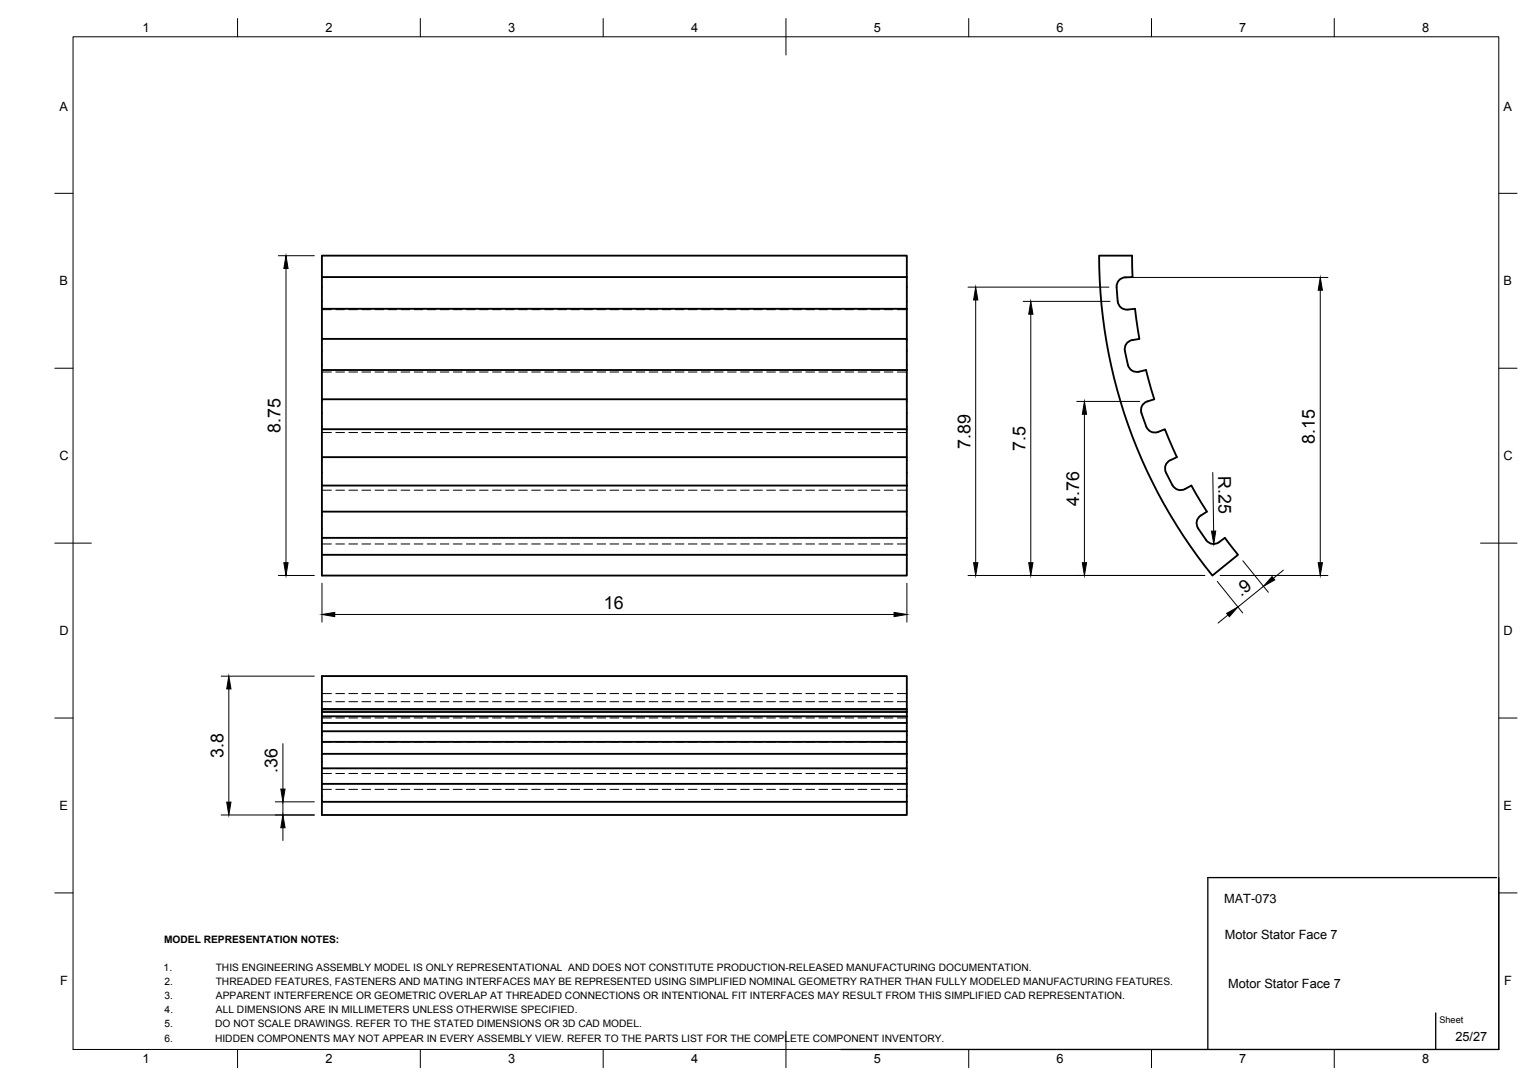
ISO-10303-21;
HEADER;
/* Generated by software containing ST-Developer
 * from STEP Tools, Inc. (www.steptools.com) 
 */

FILE_DESCRIPTION(
/* description */ ('CAx-IF Rec.Pracs.---Representation and Presentation of Product Manufa
cturing Information (PMI)---4.0---2014-10-13'),
/* implementation_level */ '2;1');

FILE_NAME(
/* name */ 'Motor Stator Face 7.step',
/* time_stamp */ '2026-10-24T18:52:33-07:00',
/* author */ (''),
/* organization */ (''),
/* preprocessor_version */ 'ST-DEVELOPER v20.2',
/* originating_system */ 'Autodesk Translation Framework v15.17.0.0',
/* authorisation */ '');

FILE_SCHEMA (('AP242_MANAGED_MODEL_BASED_3D_ENGINEERING_MIM_LF { 1 0 10303 442 2 1 4 }'));
ENDSEC;

DATA;
#10=MECHANICAL_DESIGN_GEOMETRIC_PRESENTATION_REPRESENTATION('',(#442),#34876);
#376=SHAPE_REPRESENTATION_RELATIONSHIP('SRR','None',#35013,#409);
#409=ADVANCED_BREP_SHAPE_REPRESENTATION('',(#475),#34871);
#442=STYLED_ITEM('',(#35162),#475);
#475=MANIFOLD_SOLID_BREP('Motor Stator Face 7',#19582);
#1035=PLANE('',#21978);
#1036=PLANE('',#21988);
#1037=PLANE('',#21998);
#1038=PLANE('',#22008);
#1039=PLANE('',#22018);
#1040=PLANE('',#22019);
#1041=PLANE('',#22020);
#1042=PLANE('',#22021);
#1043=PLANE('',#22022);
#1044=PLANE('',#22029);
#1045=PLANE('',#22039);
#1046=PLANE('',#22042);
#1047=PLANE('',#22045);
#1048=PLANE('',#22048);
#2531=LINE('',#33938,#4130);
#2532=LINE('',#33941,#4131);
#2533=LINE('',#33946,#4132);
#2534=LINE('',#33952,#4133);
#2535=LINE('',#33956,#4134);
#2536=LINE('',#33958,#4135);
#2537=LINE('',#33959,#4136);
#2538=LINE('',#33965,#4137);
#2539=LINE('',#33968,#4138);
#2540=LINE('',#33973,#4139);
#2541=LINE('',#33979,#4140);
#2542=LINE('',#33983,#4141);
#2543=LINE('',#33985,#4142);
#2544=LINE('',#33986,#4143);
#2545=LINE('',#33992,#4144);
#2546=LINE('',#33995,#4145);
#2547=LINE('',#34000,#4146);
#2548=LINE('',#34006,#4147);
#2549=LINE('',#34010,#4148);
#2550=LINE('',#34012,#4149);
#2551=LINE('',#34013,#4150);
#2552=LINE('',#34019,#4151);
#2553=LINE('',#34022,#4152);
#2554=LINE('',#34027,#4153);
#2555=LINE('',#34033,#4154);
#2556=LINE('',#34037,#4155);
#2557=LINE('',#34039,#4156);
#2558=LINE('',#34040,#4157);
#2559=LINE('',#34046,#4158);
#2560=LINE('',#34049,#4159);
#2561=LINE('',#34054,#4160);
#2562=LINE('',#34060,#4161);
#2563=LINE('',#34064,#4162);
#2564=LINE('',#34066,#4163);
#2565=LINE('',#34067,#4164);
#2566=LINE('',#34070,#4165);
#2567=LINE('',#34072,#4166);
#2568=LINE('',#34073,#4167);
#2569=LINE('',#34076,#4168);
#2570=LINE('',#34078,#4169);
#2571=LINE('',#34079,#4170);
#2572=LINE('',#34082,#4171);
#2573=LINE('',#34084,#4172);
#2574=LINE('',#34085,#4173);
#2575=LINE('',#34088,#4174);
#2576=LINE('',#34090,#4175);
#2577=LINE('',#34091,#4176);
#2578=LINE('',#34096,#4177);
#2579=LINE('',#34103,#4178);
#2580=LINE('',#34107,#4179);
#2581=LINE('',#34112,#4180);
#2582=LINE('',#34117,#4181);
#2583=LINE('',#34120,#4182);
#2584=LINE('',#34123,#4183);
#2585=LINE('',#34128,#4184);
#2586=LINE('',#34129,#4185);
#2587=LINE('',#34133,#4186);
#2588=LINE('',#34135,#4187);
#4130=VECTOR('',#27746,1.);
#4131=VECTOR('',#27749,1.);
#4132=VECTOR('',#27754,1.);
#4133=VECTOR('',#27761,1.);
#4134=VECTOR('',#27766,1.);
#4135=VECTOR('',#27767,1.);
#4136=VECTOR('',#27768,1.);
#4137=VECTOR('',#27773,1.);
#4138=VECTOR('',#27776,1.);
#4139=VECTOR('',#27781,1.);
#4140=VECTOR('',#27788,1.);
#4141=VECTOR('',#27793,0.999999999999999);
#4142=VECTOR('',#27794,1.);
#4143=VECTOR('',#27795,0.999999999999999);
#4144=VECTOR('',#27800,1.);
#4145=VECTOR('',#27803,1.);
#4146=VECTOR('',#27808,1.);
#4147=VECTOR('',#27815,1.);
#4148=VECTOR('',#27820,1.);
#4149=VECTOR('',#27821,1.);
#4150=VECTOR('',#27822,1.);
#4151=VECTOR('',#27827,1.);
#4152=VECTOR('',#27830,1.);
#4153=VECTOR('',#27835,1.);
#4154=VECTOR('',#27842,1.);
#4155=VECTOR('',#27847,1.);
#4156=VECTOR('',#27848,1.);
#4157=VECTOR('',#27849,1.);
#4158=VECTOR('',#27854,1.);
#4159=VECTOR('',#27857,1.);
#4160=VECTOR('',#27862,1.);
#4161=VECTOR('',#27869,1.);
#4162=VECTOR('',#27874,1.);
#4163=VECTOR('',#27875,1.);
#4164=VECTOR('',#27876,1.);
#4165=VECTOR('',#27879,1.);
#4166=VECTOR('',#27880,1.);
#4167=VECTOR('',#27881,1.);
#4168=VECTOR('',#27884,0.999999999999999);
#4169=VECTOR('',#27885,1.);
#4170=VECTOR('',#27886,0.999999999999999);
#4171=VECTOR('',#27889,1.);
#4172=VECTOR('',#27890,1.);
#4173=VECTOR('',#27891,1.);
#4174=VECTOR('',#27894,1.);
#4175=VECTOR('',#27895,1.);
#4176=VECTOR('',#27896,1.);
#4177=VECTOR('',#27901,1.);
#4178=VECTOR('',#27912,1.);
#4179=VECTOR('',#27915,1.);
#4180=VECTOR('',#27922,1.);
#4181=VECTOR('',#27929,1.);
#4182=VECTOR('',#27932,1.);
#4183=VECTOR('',#27937,1.);
#4184=VECTOR('',#27944,1.);
#4185=VECTOR('',#27945,1.);
#4186=VECTOR('',#27950,1.);
#4187=VECTOR('',#27953,1.);
#4744=CYLINDRICAL_SURFACE('',#21969,0.00025);
#4745=CYLINDRICAL_SURFACE('',#21972,0.01345);
#4746=CYLINDRICAL_SURFACE('',#21975,0.00025);
#4747=CYLINDRICAL_SURFACE('',#21979,0.00025);
#4748=CYLINDRICAL_SURFACE('',#21982,0.01345);
#4749=CYLINDRICAL_SURFACE('',#21985,0.00025);
#4750=CYLINDRICAL_SURFACE('',#21989,0.00025);
#4751=CYLINDRICAL_SURFACE('',#21992,0.01345);
#4752=CYLINDRICAL_SURFACE('',#21995,0.00025);
#4753=CYLINDRICAL_SURFACE('',#21999,0.00025);
#4754=CYLINDRICAL_SURFACE('',#22002,0.01345);
#4755=CYLINDRICAL_SURFACE('',#22005,0.00025);
#4756=CYLINDRICAL_SURFACE('',#22009,0.00025);
#4757=CYLINDRICAL_SURFACE('',#22012,0.01345);
#4758=CYLINDRICAL_SURFACE('',#22015,0.00025);
#4759=CYLINDRICAL_SURFACE('',#22023,0.013);
#4760=CYLINDRICAL_SURFACE('',#22026,0.013);
#4761=CYLINDRICAL_SURFACE('',#22035,0.013);
#4762=CYLINDRICAL_SURFACE('',#22037,0.013);
#4763=CYLINDRICAL_SURFACE('',#22040,0.013);
#4764=CYLINDRICAL_SURFACE('',#22043,0.0139);
#4765=CYLINDRICAL_SURFACE('',#22046,0.013);
#5721=FACE_OUTER_BOUND('',#6872,.T.);
#5722=FACE_OUTER_BOUND('',#6873,.T.);
#5723=FACE_OUTER_BOUND('',#6874,.T.);
#5724=FACE_OUTER_BOUND('',#6875,.T.);
#5725=FACE_OUTER_BOUND('',#6876,.T.);
#5726=FACE_OUTER_BOUND('',#6877,.T.);
#5727=FACE_OUTER_BOUND('',#6878,.T.);
#5728=FACE_OUTER_BOUND('',#6879,.T.);
#5729=FACE_OUTER_BOUND('',#6880,.T.);
#5730=FACE_OUTER_BOUND('',#6881,.T.);
#5731=FACE_OUTER_BOUND('',#6882,.T.);
#5732=FACE_OUTER_BOUND('',#6883,.T.);
#5733=FACE_OUTER_BOUND('',#6884,.T.);
#5734=FACE_OUTER_BOUND('',#6885,.T.);
#5735=FACE_OUTER_BOUND('',#6886,.T.);
#5736=FACE_OUTER_BOUND('',#6887,.T.);
#5737=FACE_OUTER_BOUND('',#6888,.T.);
#5738=FACE_OUTER_BOUND('',#6889,.T.);
#5739=FACE_OUTER_BOUND('',#6890,.T.);
#5740=FACE_OUTER_BOUND('',#6891,.T.);
#5741=FACE_OUTER_BOUND('',#6892,.T.);
#5742=FACE_OUTER_BOUND('',#6893,.T.);
#5743=FACE_OUTER_BOUND('',#6894,.T.);
#5744=FACE_OUTER_BOUND('',#6895,.T.);
#5745=FACE_OUTER_BOUND('',#6896,.T.);
#5746=FACE_OUTER_BOUND('',#6897,.T.);
#5747=FACE_OUTER_BOUND('',#6898,.T.);
#5748=FACE_OUTER_BOUND('',#6899,.T.);
#5749=FACE_OUTER_BOUND('',#6900,.T.);
#5750=FACE_OUTER_BOUND('',#6901,.T.);
#5751=FACE_OUTER_BOUND('',#6902,.T.);
#5752=FACE_OUTER_BOUND('',#6903,.T.);
#5753=FACE_OUTER_BOUND('',#6904,.T.);
#5754=FACE_OUTER_BOUND('',#6905,.T.);
#5755=FACE_OUTER_BOUND('',#6906,.T.);
#5756=FACE_OUTER_BOUND('',#6907,.T.);
#6872=EDGE_LOOP('',(#17866,#17867,#17868,#17869));
#6873=EDGE_LOOP('',(#17870,#17871,#17872,#17873));
#6874=EDGE_LOOP('',(#17874,#17875,#17876,#17877));
#6875=EDGE_LOOP('',(#17878,#17879,#17880,#17881));
#6876=EDGE_LOOP('',(#17882,#17883,#17884,#17885));
#6877=EDGE_LOOP('',(#17886,#17887,#17888,#17889));
#6878=EDGE_LOOP('',(#17890,#17891,#17892,#17893));
#6879=EDGE_LOOP('',(#17894,#17895,#17896,#17897));
#6880=EDGE_LOOP('',(#17898,#17899,#17900,#17901));
#6881=EDGE_LOOP('',(#17902,#17903,#17904,#17905));
#6882=EDGE_LOOP('',(#17906,#17907,#17908,#17909));
#6883=EDGE_LOOP('',(#17910,#17911,#17912,#17913));
#6884=EDGE_LOOP('',(#17914,#17915,#17916,#17917));
#6885=EDGE_LOOP('',(#17918,#17919,#17920,#17921));
#6886=EDGE_LOOP('',(#17922,#17923,#17924,#17925));
#6887=EDGE_LOOP('',(#17926,#17927,#17928,#17929));
#6888=EDGE_LOOP('',(#17930,#17931,#17932,#17933));
#6889=EDGE_LOOP('',(#17934,#17935,#17936,#17937));
#6890=EDGE_LOOP('',(#17938,#17939,#17940,#17941));
#6891=EDGE_LOOP('',(#17942,#17943,#17944,#17945));
#6892=EDGE_LOOP('',(#17946,#17947,#17948,#17949));
#6893=EDGE_LOOP('',(#17950,#17951,#17952,#17953));
#6894=EDGE_LOOP('',(#17954,#17955,#17956,#17957));
#6895=EDGE_LOOP('',(#17958,#17959,#17960,#17961));
#6896=EDGE_LOOP('',(#17962,#17963,#17964,#17965));
#6897=EDGE_LOOP('',(#17966,#17967,#17968,#17969));
#6898=EDGE_LOOP('',(#17970,#17971,#17972,#17973,#17974,#17975,#17976,#17977,
#17978,#17979,#17980,#17981,#17982,#17983,#17984,#17985,#17986,#17987,#17988,
#17989,#17990,#17991,#17992,#17993,#17994,#17995,#17996,#17997,#17998,#17999,
#18000,#18001,#18002,#18003));
#6899=EDGE_LOOP('',(#18004,#18005,#18006,#18007));
#6900=EDGE_LOOP('',(#18008,#18009,#18010,#18011));
#6901=EDGE_LOOP('',(#18012,#18013,#18014,#18015));
#6902=EDGE_LOOP('',(#18016,#18017,#18018,#18019));
#6903=EDGE_LOOP('',(#18020,#18021,#18022,#18023));
#6904=EDGE_LOOP('',(#18024,#18025,#18026,#18027));
#6905=EDGE_LOOP('',(#18028,#18029,#18030,#18031));
#6906=EDGE_LOOP('',(#18032,#18033,#18034,#18035));
#6907=EDGE_LOOP('',(#18036,#18037,#18038,#18039,#18040,#18041,#18042,#18043,
#18044,#18045,#18046,#18047,#18048,#18049,#18050,#18051,#18052,#18053,#18054,
#18055,#18056,#18057,#18058,#18059,#18060,#18061,#18062,#18063,#18064,#18065,
#18066,#18067,#18068,#18069));
#7941=CIRCLE('',#21970,0.000250000000012414);
#7942=CIRCLE('',#21971,0.000250000000012414);
#7943=CIRCLE('',#21973,0.0134500000000135);
#7944=CIRCLE('',#21974,0.0134500000000135);
#7945=CIRCLE('',#21976,0.000250000000012074);
#7946=CIRCLE('',#21977,0.000250000000012074);
#7947=CIRCLE('',#21980,0.000250000000011423);
#7948=CIRCLE('',#21981,0.000250000000011423);
#7949=CIRCLE('',#21983,0.0134500000000139);
#7950=CIRCLE('',#21984,0.0134500000000139);
#7951=CIRCLE('',#21986,0.00025000000001101);
#7952=CIRCLE('',#21987,0.00025000000001101);
#7953=CIRCLE('',#21990,0.000250000000010237);
#7954=CIRCLE('',#21991,0.000250000000010237);
#7955=CIRCLE('',#21993,0.0134500000000141);
#7956=CIRCLE('',#21994,0.0134500000000141);
#7957=CIRCLE('',#21996,0.000250000000010237);
#7958=CIRCLE('',#21997,0.000250000000010237);
#7959=CIRCLE('',#22000,0.00025000000001101);
#7960=CIRCLE('',#22001,0.00025000000001101);
#7961=CIRCLE('',#22003,0.0134500000000141);
#7962=CIRCLE('',#22004,0.0134500000000141);
#7963=CIRCLE('',#22006,0.000250000000011423);
#7964=CIRCLE('',#22007,0.000250000000011423);
#7965=CIRCLE('',#22010,0.000250000000012074);
#7966=CIRCLE('',#22011,0.000250000000012074);
#7967=CIRCLE('',#22013,0.0134500000000138);
#7968=CIRCLE('',#22014,0.0134500000000138);
#7969=CIRCLE('',#22016,0.000250000000012414);
#7970=CIRCLE('',#22017,0.000250000000012414);
#7971=CIRCLE('',#22024,0.0130000000000133);
#7972=CIRCLE('',#22025,0.0130000000000133);
#7973=CIRCLE('',#22027,0.0130000000000133);
#7974=CIRCLE('',#22028,0.0130000000000133);
#7975=CIRCLE('',#22030,0.0139000000000133);
#7976=CIRCLE('',#22031,0.0130000000000133);
#7977=CIRCLE('',#22032,0.0130000000000133);
#7978=CIRCLE('',#22033,0.0130000000000133);
#7979=CIRCLE('',#22034,0.0130000000000133);
#7980=CIRCLE('',#22036,0.0130000000000133);
#7981=CIRCLE('',#22038,0.0130000000000133);
#7982=CIRCLE('',#22041,0.0130000000000133);
#7983=CIRCLE('',#22044,0.0139000000000133);
#7984=CIRCLE('',#22047,0.0130000000000133);
#9751=VERTEX_POINT('',#33934);
#9752=VERTEX_POINT('',#33935);
#9753=VERTEX_POINT('',#33937);
#9754=VERTEX_POINT('',#33939);
#9755=VERTEX_POINT('',#33943);
#9756=VERTEX_POINT('',#33945);
#9757=VERTEX_POINT('',#33949);
#9758=VERTEX_POINT('',#33951);
#9759=VERTEX_POINT('',#33955);
#9760=VERTEX_POINT('',#33957);
#9761=VERTEX_POINT('',#33961);
#9762=VERTEX_POINT('',#33962);
#9763=VERTEX_POINT('',#33964);
#9764=VERTEX_POINT('',#33966);
#9765=VERTEX_POINT('',#33970);
#9766=VERTEX_POINT('',#33972);
#9767=VERTEX_POINT('',#33976);
#9768=VERTEX_POINT('',#33978);
#9769=VERTEX_POINT('',#33982);
#9770=VERTEX_POINT('',#33984);
#9771=VERTEX_POINT('',#33988);
#9772=VERTEX_POINT('',#33989);
#9773=VERTEX_POINT('',#33991);
#9774=VERTEX_POINT('',#33993);
#9775=VERTEX_POINT('',#33997);
#9776=VERTEX_POINT('',#33999);
#9777=VERTEX_POINT('',#34003);
#9778=VERTEX_POINT('',#34005);
#9779=VERTEX_POINT('',#34009);
#9780=VERTEX_POINT('',#34011);
#9781=VERTEX_POINT('',#34015);
#9782=VERTEX_POINT('',#34016);
#9783=VERTEX_POINT('',#34018);
#9784=VERTEX_POINT('',#34020);
#9785=VERTEX_POINT('',#34024);
#9786=VERTEX_POINT('',#34026);
#9787=VERTEX_POINT('',#34030);
#9788=VERTEX_POINT('',#34032);
#9789=VERTEX_POINT('',#34036);
#9790=VERTEX_POINT('',#34038);
#9791=VERTEX_POINT('',#34042);
#9792=VERTEX_POINT('',#34043);
#9793=VERTEX_POINT('',#34045);
#9794=VERTEX_POINT('',#34047);
#9795=VERTEX_POINT('',#34051);
#9796=VERTEX_POINT('',#34053);
#9797=VERTEX_POINT('',#34057);
#9798=VERTEX_POINT('',#34059);
#9799=VERTEX_POINT('',#34063);
#9800=VERTEX_POINT('',#34065);
#9801=VERTEX_POINT('',#34069);
#9802=VERTEX_POINT('',#34071);
#9803=VERTEX_POINT('',#34075);
#9804=VERTEX_POINT('',#34077);
#9805=VERTEX_POINT('',#34081);
#9806=VERTEX_POINT('',#34083);
#9807=VERTEX_POINT('',#34087);
#9808=VERTEX_POINT('',#34089);
#9809=VERTEX_POINT('',#34093);
#9810=VERTEX_POINT('',#34095);
#9811=VERTEX_POINT('',#34102);
#9812=VERTEX_POINT('',#34104);
#9813=VERTEX_POINT('',#34106);
#9814=VERTEX_POINT('',#34110);
#9815=VERTEX_POINT('',#34115);
#9816=VERTEX_POINT('',#34119);
#9817=VERTEX_POINT('',#34127);
#9818=VERTEX_POINT('',#34131);
#12491=EDGE_CURVE('',#9751,#9752,#7941,.T.);
#12492=EDGE_CURVE('',#9752,#9753,#2531,.T.);
#12493=EDGE_CURVE('',#9753,#9754,#7942,.T.);
#12494=EDGE_CURVE('',#9754,#9751,#2532,.T.);
#12495=EDGE_CURVE('',#9755,#9752,#7943,.T.);
#12496=EDGE_CURVE('',#9756,#9755,#2533,.T.);
#12497=EDGE_CURVE('',#9753,#9756,#7944,.T.);
#12498=EDGE_CURVE('',#9755,#9757,#7945,.T.);
#12499=EDGE_CURVE('',#9757,#9758,#2534,.T.);
#12500=EDGE_CURVE('',#9758,#9756,#7946,.T.);
#12501=EDGE_CURVE('',#9759,#9757,#2535,.T.);
#12502=EDGE_CURVE('',#9760,#9759,#2536,.T.);
#12503=EDGE_CURVE('',#9758,#9760,#2537,.T.);
#12504=EDGE_CURVE('',#9761,#9762,#7947,.T.);
#12505=EDGE_CURVE('',#9762,#9763,#2538,.T.);
#12506=EDGE_CURVE('',#9763,#9764,#7948,.T.);
#12507=EDGE_CURVE('',#9764,#9761,#2539,.T.);
#12508=EDGE_CURVE('',#9765,#9762,#7949,.T.);
#12509=EDGE_CURVE('',#9766,#9765,#2540,.T.);
#12510=EDGE_CURVE('',#9763,#9766,#7950,.T.);
#12511=EDGE_CURVE('',#9765,#9767,#7951,.T.);
#12512=EDGE_CURVE('',#9767,#9768,#2541,.T.);
#12513=EDGE_CURVE('',#9768,#9766,#7952,.T.);
#12514=EDGE_CURVE('',#9769,#9767,#2542,.T.);
#12515=EDGE_CURVE('',#9770,#9769,#2543,.T.);
#12516=EDGE_CURVE('',#9768,#9770,#2544,.T.);
#12517=EDGE_CURVE('',#9771,#9772,#7953,.T.);
#12518=EDGE_CURVE('',#9772,#9773,#2545,.T.);
#12519=EDGE_CURVE('',#9773,#9774,#7954,.T.);
#12520=EDGE_CURVE('',#9774,#9771,#2546,.T.);
#12521=EDGE_CURVE('',#9775,#9772,#7955,.T.);
#12522=EDGE_CURVE('',#9776,#9775,#2547,.T.);
#12523=EDGE_CURVE('',#9773,#9776,#7956,.T.);
#12524=EDGE_CURVE('',#9775,#9777,#7957,.T.);
#12525=EDGE_CURVE('',#9777,#9778,#2548,.T.);
#12526=EDGE_CURVE('',#9778,#9776,#7958,.T.);
#12527=EDGE_CURVE('',#9779,#9777,#2549,.T.);
#12528=EDGE_CURVE('',#9780,#9779,#2550,.T.);
#12529=EDGE_CURVE('',#9778,#9780,#2551,.T.);
#12530=EDGE_CURVE('',#9781,#9782,#7959,.T.);
#12531=EDGE_CURVE('',#9782,#9783,#2552,.T.);
#12532=EDGE_CURVE('',#9783,#9784,#7960,.T.);
#12533=EDGE_CURVE('',#9784,#9781,#2553,.T.);
#12534=EDGE_CURVE('',#9785,#9782,#7961,.T.);
#12535=EDGE_CURVE('',#9786,#9785,#2554,.T.);
#12536=EDGE_CURVE('',#9783,#9786,#7962,.T.);
#12537=EDGE_CURVE('',#9785,#9787,#7963,.T.);
#12538=EDGE_CURVE('',#9787,#9788,#2555,.T.);
#12539=EDGE_CURVE('',#9788,#9786,#7964,.T.);
#12540=EDGE_CURVE('',#9789,#9787,#2556,.T.);
#12541=EDGE_CURVE('',#9790,#9789,#2557,.T.);
#12542=EDGE_CURVE('',#9788,#9790,#2558,.T.);
#12543=EDGE_CURVE('',#9791,#9792,#7965,.T.);
#12544=EDGE_CURVE('',#9792,#9793,#2559,.T.);
#12545=EDGE_CURVE('',#9793,#9794,#7966,.T.);
#12546=EDGE_CURVE('',#9794,#9791,#2560,.T.);
#12547=EDGE_CURVE('',#9795,#9792,#7967,.T.);
#12548=EDGE_CURVE('',#9796,#9795,#2561,.T.);
#12549=EDGE_CURVE('',#9793,#9796,#7968,.T.);
#12550=EDGE_CURVE('',#9795,#9797,#7969,.T.);
#12551=EDGE_CURVE('',#9797,#9798,#2562,.T.);
#12552=EDGE_CURVE('',#9798,#9796,#7970,.T.);
#12553=EDGE_CURVE('',#9799,#9797,#2563,.T.);
#12554=EDGE_CURVE('',#9800,#9799,#2564,.T.);
#12555=EDGE_CURVE('',#9798,#9800,#2565,.T.);
#12556=EDGE_CURVE('',#9801,#9794,#2566,.T.);
#12557=EDGE_CURVE('',#9802,#9801,#2567,.T.);
#12558=EDGE_CURVE('',#9791,#9802,#2568,.T.);
#12559=EDGE_CURVE('',#9803,#9784,#2569,.T.);
#12560=EDGE_CURVE('',#9804,#9803,#2570,.T.);
#12561=EDGE_CURVE('',#9781,#9804,#2571,.T.);
#12562=EDGE_CURVE('',#9805,#9764,#2572,.T.);
#12563=EDGE_CURVE('',#9806,#9805,#2573,.T.);
#12564=EDGE_CURVE('',#9761,#9806,#2574,.T.);
#12565=EDGE_CURVE('',#9807,#9754,#2575,.T.);
#12566=EDGE_CURVE('',#9808,#9807,#2576,.T.);
#12567=EDGE_CURVE('',#9751,#9808,#2577,.T.);
#12568=EDGE_CURVE('',#9809,#9799,#7971,.T.);
#12569=EDGE_CURVE('',#9809,#9810,#2578,.T.);
#12570=EDGE_CURVE('',#9800,#9810,#7972,.T.);
#12571=EDGE_CURVE('',#9780,#9803,#7973,.T.);
#12572=EDGE_CURVE('',#9804,#9779,#7974,.T.);
#12573=EDGE_CURVE('',#9810,#9811,#2579,.T.);
#12574=EDGE_CURVE('',#9811,#9812,#7975,.T.);
#12575=EDGE_CURVE('',#9812,#9813,#2580,.T.);
#12576=EDGE_CURVE('',#9813,#9807,#7976,.T.);
#12577=EDGE_CURVE('',#9760,#9805,#7977,.T.);
#12578=EDGE_CURVE('',#9770,#9814,#7978,.T.);
#12579=EDGE_CURVE('',#9814,#9774,#2581,.T.);
#12580=EDGE_CURVE('',#9790,#9801,#7979,.T.);
#12581=EDGE_CURVE('',#9815,#9769,#7980,.T.);
#12582=EDGE_CURVE('',#9815,#9814,#2582,.T.);
#12583=EDGE_CURVE('',#9813,#9816,#2583,.T.);
#12584=EDGE_CURVE('',#9808,#9816,#7981,.T.);
#12585=EDGE_CURVE('',#9771,#9815,#2584,.T.);
#12586=EDGE_CURVE('',#9802,#9789,#7982,.T.);
#12587=EDGE_CURVE('',#9817,#9809,#2585,.T.);
#12588=EDGE_CURVE('',#9811,#9817,#2586,.T.);
#12589=EDGE_CURVE('',#9818,#9817,#7983,.T.);
#12590=EDGE_CURVE('',#9812,#9818,#2587,.T.);
#12591=EDGE_CURVE('',#9816,#9818,#2588,.T.);
#12592=EDGE_CURVE('',#9806,#9759,#7984,.T.);
#17866=ORIENTED_EDGE('',*,*,#12491,.T.);
#17867=ORIENTED_EDGE('',*,*,#12492,.T.);
#17868=ORIENTED_EDGE('',*,*,#12493,.T.);
#17869=ORIENTED_EDGE('',*,*,#12494,.T.);
#17870=ORIENTED_EDGE('',*,*,#12492,.F.);
#17871=ORIENTED_EDGE('',*,*,#12495,.F.);
#17872=ORIENTED_EDGE('',*,*,#12496,.F.);
#17873=ORIENTED_EDGE('',*,*,#12497,.F.);
#17874=ORIENTED_EDGE('',*,*,#12498,.T.);
#17875=ORIENTED_EDGE('',*,*,#12499,.T.);
#17876=ORIENTED_EDGE('',*,*,#12500,.T.);
#17877=ORIENTED_EDGE('',*,*,#12496,.T.);
#17878=ORIENTED_EDGE('',*,*,#12499,.F.);
#17879=ORIENTED_EDGE('',*,*,#12501,.F.);
#17880=ORIENTED_EDGE('',*,*,#12502,.F.);
#17881=ORIENTED_EDGE('',*,*,#12503,.F.);
#17882=ORIENTED_EDGE('',*,*,#12504,.T.);
#17883=ORIENTED_EDGE('',*,*,#12505,.T.);
#17884=ORIENTED_EDGE('',*,*,#12506,.T.);
#17885=ORIENTED_EDGE('',*,*,#12507,.T.);
#17886=ORIENTED_EDGE('',*,*,#12505,.F.);
#17887=ORIENTED_EDGE('',*,*,#12508,.F.);
#17888=ORIENTED_EDGE('',*,*,#12509,.F.);
#17889=ORIENTED_EDGE('',*,*,#12510,.F.);
#17890=ORIENTED_EDGE('',*,*,#12511,.T.);
#17891=ORIENTED_EDGE('',*,*,#12512,.T.);
#17892=ORIENTED_EDGE('',*,*,#12513,.T.);
#17893=ORIENTED_EDGE('',*,*,#12509,.T.);
#17894=ORIENTED_EDGE('',*,*,#12512,.F.);
#17895=ORIENTED_EDGE('',*,*,#12514,.F.);
#17896=ORIENTED_EDGE('',*,*,#12515,.F.);
#17897=ORIENTED_EDGE('',*,*,#12516,.F.);
#17898=ORIENTED_EDGE('',*,*,#12517,.T.);
#17899=ORIENTED_EDGE('',*,*,#12518,.T.);
#17900=ORIENTED_EDGE('',*,*,#12519,.T.);
#17901=ORIENTED_EDGE('',*,*,#12520,.T.);
#17902=ORIENTED_EDGE('',*,*,#12518,.F.);
#17903=ORIENTED_EDGE('',*,*,#12521,.F.);
#17904=ORIENTED_EDGE('',*,*,#12522,.F.);
#17905=ORIENTED_EDGE('',*,*,#12523,.F.);
#17906=ORIENTED_EDGE('',*,*,#12524,.T.);
#17907=ORIENTED_EDGE('',*,*,#12525,.T.);
#17908=ORIENTED_EDGE('',*,*,#12526,.T.);
#17909=ORIENTED_EDGE('',*,*,#12522,.T.);
#17910=ORIENTED_EDGE('',*,*,#12525,.F.);
#17911=ORIENTED_EDGE('',*,*,#12527,.F.);
#17912=ORIENTED_EDGE('',*,*,#12528,.F.);
#17913=ORIENTED_EDGE('',*,*,#12529,.F.);
#17914=ORIENTED_EDGE('',*,*,#12530,.T.);
#17915=ORIENTED_EDGE('',*,*,#12531,.T.);
#17916=ORIENTED_EDGE('',*,*,#12532,.T.);
#17917=ORIENTED_EDGE('',*,*,#12533,.T.);
#17918=ORIENTED_EDGE('',*,*,#12531,.F.);
#17919=ORIENTED_EDGE('',*,*,#12534,.F.);
#17920=ORIENTED_EDGE('',*,*,#12535,.F.);
#17921=ORIENTED_EDGE('',*,*,#12536,.F.);
#17922=ORIENTED_EDGE('',*,*,#12537,.T.);
#17923=ORIENTED_EDGE('',*,*,#12538,.T.);
#17924=ORIENTED_EDGE('',*,*,#12539,.T.);
#17925=ORIENTED_EDGE('',*,*,#12535,.T.);
#17926=ORIENTED_EDGE('',*,*,#12538,.F.);
#17927=ORIENTED_EDGE('',*,*,#12540,.F.);
#17928=ORIENTED_EDGE('',*,*,#12541,.F.);
#17929=ORIENTED_EDGE('',*,*,#12542,.F.);
#17930=ORIENTED_EDGE('',*,*,#12543,.T.);
#17931=ORIENTED_EDGE('',*,*,#12544,.T.);
#17932=ORIENTED_EDGE('',*,*,#12545,.T.);
#17933=ORIENTED_EDGE('',*,*,#12546,.T.);
#17934=ORIENTED_EDGE('',*,*,#12544,.F.);
#17935=ORIENTED_EDGE('',*,*,#12547,.F.);
#17936=ORIENTED_EDGE('',*,*,#12548,.F.);
#17937=ORIENTED_EDGE('',*,*,#12549,.F.);
#17938=ORIENTED_EDGE('',*,*,#12550,.T.);
#17939=ORIENTED_EDGE('',*,*,#12551,.T.);
#17940=ORIENTED_EDGE('',*,*,#12552,.T.);
#17941=ORIENTED_EDGE('',*,*,#12548,.T.);
#17942=ORIENTED_EDGE('',*,*,#12551,.F.);
#17943=ORIENTED_EDGE('',*,*,#12553,.F.);
#17944=ORIENTED_EDGE('',*,*,#12554,.F.);
#17945=ORIENTED_EDGE('',*,*,#12555,.F.);
#17946=ORIENTED_EDGE('',*,*,#12546,.F.);
#17947=ORIENTED_EDGE('',*,*,#12556,.F.);
#17948=ORIENTED_EDGE('',*,*,#12557,.F.);
#17949=ORIENTED_EDGE('',*,*,#12558,.F.);
#17950=ORIENTED_EDGE('',*,*,#12533,.F.);
#17951=ORIENTED_EDGE('',*,*,#12559,.F.);
#17952=ORIENTED_EDGE('',*,*,#12560,.F.);
#17953=ORIENTED_EDGE('',*,*,#12561,.F.);
#17954=ORIENTED_EDGE('',*,*,#12507,.F.);
#17955=ORIENTED_EDGE('',*,*,#12562,.F.);
#17956=ORIENTED_EDGE('',*,*,#12563,.F.);
#17957=ORIENTED_EDGE('',*,*,#12564,.F.);
#17958=ORIENTED_EDGE('',*,*,#12494,.F.);
#17959=ORIENTED_EDGE('',*,*,#12565,.F.);
#17960=ORIENTED_EDGE('',*,*,#12566,.F.);
#17961=ORIENTED_EDGE('',*,*,#12567,.F.);
#17962=ORIENTED_EDGE('',*,*,#12554,.T.);
#17963=ORIENTED_EDGE('',*,*,#12568,.F.);
#17964=ORIENTED_EDGE('',*,*,#12569,.T.);
#17965=ORIENTED_EDGE('',*,*,#12570,.F.);
#17966=ORIENTED_EDGE('',*,*,#12560,.T.);
#17967=ORIENTED_EDGE('',*,*,#12571,.F.);
#17968=ORIENTED_EDGE('',*,*,#12528,.T.);
#17969=ORIENTED_EDGE('',*,*,#12572,.F.);
#17970=ORIENTED_EDGE('',*,*,#12556,.T.);
#17971=ORIENTED_EDGE('',*,*,#12545,.F.);
#17972=ORIENTED_EDGE('',*,*,#12549,.T.);
#17973=ORIENTED_EDGE('',*,*,#12552,.F.);
#17974=ORIENTED_EDGE('',*,*,#12555,.T.);
#17975=ORIENTED_EDGE('',*,*,#12570,.T.);
#17976=ORIENTED_EDGE('',*,*,#12573,.T.);
#17977=ORIENTED_EDGE('',*,*,#12574,.T.);
#17978=ORIENTED_EDGE('',*,*,#12575,.T.);
#17979=ORIENTED_EDGE('',*,*,#12576,.T.);
#17980=ORIENTED_EDGE('',*,*,#12565,.T.);
#17981=ORIENTED_EDGE('',*,*,#12493,.F.);
#17982=ORIENTED_EDGE('',*,*,#12497,.T.);
#17983=ORIENTED_EDGE('',*,*,#12500,.F.);
#17984=ORIENTED_EDGE('',*,*,#12503,.T.);
#17985=ORIENTED_EDGE('',*,*,#12577,.T.);
#17986=ORIENTED_EDGE('',*,*,#12562,.T.);
#17987=ORIENTED_EDGE('',*,*,#12506,.F.);
#17988=ORIENTED_EDGE('',*,*,#12510,.T.);
#17989=ORIENTED_EDGE('',*,*,#12513,.F.);
#17990=ORIENTED_EDGE('',*,*,#12516,.T.);
#17991=ORIENTED_EDGE('',*,*,#12578,.T.);
#17992=ORIENTED_EDGE('',*,*,#12579,.T.);
#17993=ORIENTED_EDGE('',*,*,#12519,.F.);
#17994=ORIENTED_EDGE('',*,*,#12523,.T.);
#17995=ORIENTED_EDGE('',*,*,#12526,.F.);
#17996=ORIENTED_EDGE('',*,*,#12529,.T.);
#17997=ORIENTED_EDGE('',*,*,#12571,.T.);
#17998=ORIENTED_EDGE('',*,*,#12559,.T.);
#17999=ORIENTED_EDGE('',*,*,#12532,.F.);
#18000=ORIENTED_EDGE('',*,*,#12536,.T.);
#18001=ORIENTED_EDGE('',*,*,#12539,.F.);
#18002=ORIENTED_EDGE('',*,*,#12542,.T.);
#18003=ORIENTED_EDGE('',*,*,#12580,.T.);
#18004=ORIENTED_EDGE('',*,*,#12515,.T.);
#18005=ORIENTED_EDGE('',*,*,#12581,.F.);
#18006=ORIENTED_EDGE('',*,*,#12582,.T.);
#18007=ORIENTED_EDGE('',*,*,#12578,.F.);
#18008=ORIENTED_EDGE('',*,*,#12566,.T.);
#18009=ORIENTED_EDGE('',*,*,#12576,.F.);
#18010=ORIENTED_EDGE('',*,*,#12583,.T.);
#18011=ORIENTED_EDGE('',*,*,#12584,.F.);
#18012=ORIENTED_EDGE('',*,*,#12520,.F.);
#18013=ORIENTED_EDGE('',*,*,#12579,.F.);
#18014=ORIENTED_EDGE('',*,*,#12582,.F.);
#18015=ORIENTED_EDGE('',*,*,#12585,.F.);
#18016=ORIENTED_EDGE('',*,*,#12557,.T.);
#18017=ORIENTED_EDGE('',*,*,#12580,.F.);
#18018=ORIENTED_EDGE('',*,*,#12541,.T.);
#18019=ORIENTED_EDGE('',*,*,#12586,.F.);
#18020=ORIENTED_EDGE('',*,*,#12569,.F.);
#18021=ORIENTED_EDGE('',*,*,#12587,.F.);
#18022=ORIENTED_EDGE('',*,*,#12588,.F.);
#18023=ORIENTED_EDGE('',*,*,#12573,.F.);
#18024=ORIENTED_EDGE('',*,*,#12588,.T.);
#18025=ORIENTED_EDGE('',*,*,#12589,.F.);
#18026=ORIENTED_EDGE('',*,*,#12590,.F.);
#18027=ORIENTED_EDGE('',*,*,#12574,.F.);
#18028=ORIENTED_EDGE('',*,*,#12590,.T.);
#18029=ORIENTED_EDGE('',*,*,#12591,.F.);
#18030=ORIENTED_EDGE('',*,*,#12583,.F.);
#18031=ORIENTED_EDGE('',*,*,#12575,.F.);
#18032=ORIENTED_EDGE('',*,*,#12563,.T.);
#18033=ORIENTED_EDGE('',*,*,#12577,.F.);
#18034=ORIENTED_EDGE('',*,*,#12502,.T.);
#18035=ORIENTED_EDGE('',*,*,#12592,.F.);
#18036=ORIENTED_EDGE('',*,*,#12558,.T.);
#18037=ORIENTED_EDGE('',*,*,#12586,.T.);
#18038=ORIENTED_EDGE('',*,*,#12540,.T.);
#18039=ORIENTED_EDGE('',*,*,#12537,.F.);
#18040=ORIENTED_EDGE('',*,*,#12534,.T.);
#18041=ORIENTED_EDGE('',*,*,#12530,.F.);
#18042=ORIENTED_EDGE('',*,*,#12561,.T.);
#18043=ORIENTED_EDGE('',*,*,#12572,.T.);
#18044=ORIENTED_EDGE('',*,*,#12527,.T.);
#18045=ORIENTED_EDGE('',*,*,#12524,.F.);
#18046=ORIENTED_EDGE('',*,*,#12521,.T.);
#18047=ORIENTED_EDGE('',*,*,#12517,.F.);
#18048=ORIENTED_EDGE('',*,*,#12585,.T.);
#18049=ORIENTED_EDGE('',*,*,#12581,.T.);
#18050=ORIENTED_EDGE('',*,*,#12514,.T.);
#18051=ORIENTED_EDGE('',*,*,#12511,.F.);
#18052=ORIENTED_EDGE('',*,*,#12508,.T.);
#18053=ORIENTED_EDGE('',*,*,#12504,.F.);
#18054=ORIENTED_EDGE('',*,*,#12564,.T.);
#18055=ORIENTED_EDGE('',*,*,#12592,.T.);
#18056=ORIENTED_EDGE('',*,*,#12501,.T.);
#18057=ORIENTED_EDGE('',*,*,#12498,.F.);
#18058=ORIENTED_EDGE('',*,*,#12495,.T.);
#18059=ORIENTED_EDGE('',*,*,#12491,.F.);
#18060=ORIENTED_EDGE('',*,*,#12567,.T.);
#18061=ORIENTED_EDGE('',*,*,#12584,.T.);
#18062=ORIENTED_EDGE('',*,*,#12591,.T.);
#18063=ORIENTED_EDGE('',*,*,#12589,.T.);
#18064=ORIENTED_EDGE('',*,*,#12587,.T.);
#18065=ORIENTED_EDGE('',*,*,#12568,.T.);
#18066=ORIENTED_EDGE('',*,*,#12553,.T.);
#18067=ORIENTED_EDGE('',*,*,#12550,.F.);
#18068=ORIENTED_EDGE('',*,*,#12547,.T.);
#18069=ORIENTED_EDGE('',*,*,#12543,.F.);
#19437=ADVANCED_FACE('',(#5721),#4744,.F.);
#19438=ADVANCED_FACE('',(#5722),#4745,.F.);
#19439=ADVANCED_FACE('',(#5723),#4746,.F.);
#19440=ADVANCED_FACE('',(#5724),#1035,.F.);
#19441=ADVANCED_FACE('',(#5725),#4747,.F.);
#19442=ADVANCED_FACE('',(#5726),#4748,.F.);
#19443=ADVANCED_FACE('',(#5727),#4749,.F.);
#19444=ADVANCED_FACE('',(#5728),#1036,.F.);
#19445=ADVANCED_FACE('',(#5729),#4750,.F.);
#19446=ADVANCED_FACE('',(#5730),#4751,.F.);
#19447=ADVANCED_FACE('',(#5731),#4752,.F.);
#19448=ADVANCED_FACE('',(#5732),#1037,.F.);
#19449=ADVANCED_FACE('',(#5733),#4753,.F.);
#19450=ADVANCED_FACE('',(#5734),#4754,.F.);
#19451=ADVANCED_FACE('',(#5735),#4755,.F.);
#19452=ADVANCED_FACE('',(#5736),#1038,.F.);
#19453=ADVANCED_FACE('',(#5737),#4756,.F.);
#19454=ADVANCED_FACE('',(#5738),#4757,.F.);
#19455=ADVANCED_FACE('',(#5739),#4758,.F.);
#19456=ADVANCED_FACE('',(#5740),#1039,.F.);
#19457=ADVANCED_FACE('',(#5741),#1040,.F.);
#19458=ADVANCED_FACE('',(#5742),#1041,.F.);
#19459=ADVANCED_FACE('',(#5743),#1042,.F.);
#19460=ADVANCED_FACE('',(#5744),#1043,.F.);
#19461=ADVANCED_FACE('',(#5745),#4759,.F.);
#19462=ADVANCED_FACE('',(#5746),#4760,.F.);
#19463=ADVANCED_FACE('',(#5747),#1044,.F.);
#19464=ADVANCED_FACE('',(#5748),#4761,.F.);
#19465=ADVANCED_FACE('',(#5749),#4762,.F.);
#19466=ADVANCED_FACE('',(#5750),#1045,.F.);
#19467=ADVANCED_FACE('',(#5751),#4763,.F.);
#19468=ADVANCED_FACE('',(#5752),#1046,.T.);
#19469=ADVANCED_FACE('',(#5753),#4764,.T.);
#19470=ADVANCED_FACE('',(#5754),#1047,.T.);
#19471=ADVANCED_FACE('',(#5755),#4765,.F.);
#19472=ADVANCED_FACE('',(#5756),#1048,.T.);
#19582=CLOSED_SHELL('',(#19437,#19438,#19439,#19440,#19441,#19442,#19443,
#19444,#19445,#19446,#19447,#19448,#19449,#19450,#19451,#19452,#19453,#19454,
#19455,#19456,#19457,#19458,#19459,#19460,#19461,#19462,#19463,#19464,#19465,
#19466,#19467,#19468,#19469,#19470,#19471,#19472));
#21968=AXIS2_PLACEMENT_3D('',#33932,#27740,#27741);
#21969=AXIS2_PLACEMENT_3D('',#33933,#27742,#27743);
#21970=AXIS2_PLACEMENT_3D('',#33936,#27744,#27745);
#21971=AXIS2_PLACEMENT_3D('',#33940,#27747,#27748);
#21972=AXIS2_PLACEMENT_3D('',#33942,#27750,#27751);
#21973=AXIS2_PLACEMENT_3D('',#33944,#27752,#27753);
#21974=AXIS2_PLACEMENT_3D('',#33947,#27755,#27756);
#21975=AXIS2_PLACEMENT_3D('',#33948,#27757,#27758);
#21976=AXIS2_PLACEMENT_3D('',#33950,#27759,#27760);
#21977=AXIS2_PLACEMENT_3D('',#33953,#27762,#27763);
#21978=AXIS2_PLACEMENT_3D('',#33954,#27764,#27765);
#21979=AXIS2_PLACEMENT_3D('',#33960,#27769,#27770);
#21980=AXIS2_PLACEMENT_3D('',#33963,#27771,#27772);
#21981=AXIS2_PLACEMENT_3D('',#33967,#27774,#27775);
#21982=AXIS2_PLACEMENT_3D('',#33969,#27777,#27778);
#21983=AXIS2_PLACEMENT_3D('',#33971,#27779,#27780);
#21984=AXIS2_PLACEMENT_3D('',#33974,#27782,#27783);
#21985=AXIS2_PLACEMENT_3D('',#33975,#27784,#27785);
#21986=AXIS2_PLACEMENT_3D('',#33977,#27786,#27787);
#21987=AXIS2_PLACEMENT_3D('',#33980,#27789,#27790);
#21988=AXIS2_PLACEMENT_3D('',#33981,#27791,#27792);
#21989=AXIS2_PLACEMENT_3D('',#33987,#27796,#27797);
#21990=AXIS2_PLACEMENT_3D('',#33990,#27798,#27799);
#21991=AXIS2_PLACEMENT_3D('',#33994,#27801,#27802);
#21992=AXIS2_PLACEMENT_3D('',#33996,#27804,#27805);
#21993=AXIS2_PLACEMENT_3D('',#33998,#27806,#27807);
#21994=AXIS2_PLACEMENT_3D('',#34001,#27809,#27810);
#21995=AXIS2_PLACEMENT_3D('',#34002,#27811,#27812);
#21996=AXIS2_PLACEMENT_3D('',#34004,#27813,#27814);
#21997=AXIS2_PLACEMENT_3D('',#34007,#27816,#27817);
#21998=AXIS2_PLACEMENT_3D('',#34008,#27818,#27819);
#21999=AXIS2_PLACEMENT_3D('',#34014,#27823,#27824);
#22000=AXIS2_PLACEMENT_3D('',#34017,#27825,#27826);
#22001=AXIS2_PLACEMENT_3D('',#34021,#27828,#27829);
#22002=AXIS2_PLACEMENT_3D('',#34023,#27831,#27832);
#22003=AXIS2_PLACEMENT_3D('',#34025,#27833,#27834);
#22004=AXIS2_PLACEMENT_3D('',#34028,#27836,#27837);
#22005=AXIS2_PLACEMENT_3D('',#34029,#27838,#27839);
#22006=AXIS2_PLACEMENT_3D('',#34031,#27840,#27841);
#22007=AXIS2_PLACEMENT_3D('',#34034,#27843,#27844);
#22008=AXIS2_PLACEMENT_3D('',#34035,#27845,#27846);
#22009=AXIS2_PLACEMENT_3D('',#34041,#27850,#27851);
#22010=AXIS2_PLACEMENT_3D('',#34044,#27852,#27853);
#22011=AXIS2_PLACEMENT_3D('',#34048,#27855,#27856);
#22012=AXIS2_PLACEMENT_3D('',#34050,#27858,#27859);
#22013=AXIS2_PLACEMENT_3D('',#34052,#27860,#27861);
#22014=AXIS2_PLACEMENT_3D('',#34055,#27863,#27864);
#22015=AXIS2_PLACEMENT_3D('',#34056,#27865,#27866);
#22016=AXIS2_PLACEMENT_3D('',#34058,#27867,#27868);
#22017=AXIS2_PLACEMENT_3D('',#34061,#27870,#27871);
#22018=AXIS2_PLACEMENT_3D('',#34062,#27872,#27873);
#22019=AXIS2_PLACEMENT_3D('',#34068,#27877,#27878);
#22020=AXIS2_PLACEMENT_3D('',#34074,#27882,#27883);
#22021=AXIS2_PLACEMENT_3D('',#34080,#27887,#27888);
#22022=AXIS2_PLACEMENT_3D('',#34086,#27892,#27893);
#22023=AXIS2_PLACEMENT_3D('',#34092,#27897,#27898);
#22024=AXIS2_PLACEMENT_3D('',#34094,#27899,#27900);
#22025=AXIS2_PLACEMENT_3D('',#34097,#27902,#27903);
#22026=AXIS2_PLACEMENT_3D('',#34098,#27904,#27905);
#22027=AXIS2_PLACEMENT_3D('',#34099,#27906,#27907);
#22028=AXIS2_PLACEMENT_3D('',#34100,#27908,#27909);
#22029=AXIS2_PLACEMENT_3D('',#34101,#27910,#27911);
#22030=AXIS2_PLACEMENT_3D('',#34105,#27913,#27914);
#22031=AXIS2_PLACEMENT_3D('',#34108,#27916,#27917);
#22032=AXIS2_PLACEMENT_3D('',#34109,#27918,#27919);
#22033=AXIS2_PLACEMENT_3D('',#34111,#27920,#27921);
#22034=AXIS2_PLACEMENT_3D('',#34113,#27923,#27924);
#22035=AXIS2_PLACEMENT_3D('',#34114,#27925,#27926);
#22036=AXIS2_PLACEMENT_3D('',#34116,#27927,#27928);
#22037=AXIS2_PLACEMENT_3D('',#34118,#27930,#27931);
#22038=AXIS2_PLACEMENT_3D('',#34121,#27933,#27934);
#22039=AXIS2_PLACEMENT_3D('',#34122,#27935,#27936);
#22040=AXIS2_PLACEMENT_3D('',#34124,#27938,#27939);
#22041=AXIS2_PLACEMENT_3D('',#34125,#27940,#27941);
#22042=AXIS2_PLACEMENT_3D('',#34126,#27942,#27943);
#22043=AXIS2_PLACEMENT_3D('',#34130,#27946,#27947);
#22044=AXIS2_PLACEMENT_3D('',#34132,#27948,#27949);
#22045=AXIS2_PLACEMENT_3D('',#34134,#27951,#27952);
#22046=AXIS2_PLACEMENT_3D('',#34136,#27954,#27955);
#22047=AXIS2_PLACEMENT_3D('',#34137,#27956,#27957);
#22048=AXIS2_PLACEMENT_3D('',#34138,#27958,#27959);
#27740=DIRECTION('axis',(0.,0.,1.));
#27741=DIRECTION('refdir',(1.,0.,0.));
#27742=DIRECTION('center_axis',(0.,-1.,0.));
#27743=DIRECTION('ref_axis',(-0.281918008728671,0.,0.95943850055877));
#27744=DIRECTION('center_axis',(0.,1.,0.));
#27745=DIRECTION('ref_axis',(-0.281918008754672,0.,0.95943850055113));
#27746=DIRECTION('',(0.,-1.,0.));
#27747=DIRECTION('center_axis',(0.,-1.,0.));
#27748=DIRECTION('ref_axis',(-0.281918008754672,0.,0.95943850055113));
#27749=DIRECTION('',(0.,1.,0.));
#27750=DIRECTION('center_axis',(0.,-1.,0.));
#27751=DIRECTION('ref_axis',(0.470745247127108,0.,0.882269183586981));
#27752=DIRECTION('center_axis',(0.,-1.,0.));
#27753=DIRECTION('ref_axis',(0.470745247127378,0.,0.882269183586837));
#27754=DIRECTION('',(0.,1.,0.));
#27755=DIRECTION('center_axis',(0.,1.,0.));
#27756=DIRECTION('ref_axis',(0.470745247127378,0.,0.882269183586837));
#27757=DIRECTION('center_axis',(0.,-1.,0.));
#27758=DIRECTION('ref_axis',(0.971857119217081,0.,0.235571092936032));
#27759=DIRECTION('center_axis',(0.,1.,0.));
#27760=DIRECTION('ref_axis',(0.971857119210143,0.,0.235571092964655));
#27761=DIRECTION('',(0.,-1.,0.));
#27762=DIRECTION('center_axis',(0.,-1.,0.));
#27763=DIRECTION('ref_axis',(0.971857119210143,0.,0.235571092964655));
#27764=DIRECTION('center_axis',(0.848811934516349,0.,-0.528694902398929));
#27765=DIRECTION('ref_axis',(0.,-1.,0.));
#27766=DIRECTION('',(0.528694902399201,0.,0.84881193451618));
#27767=DIRECTION('',(0.,1.,0.));
#27768=DIRECTION('',(-0.528694902399201,0.,-0.84881193451618));
#27769=DIRECTION('center_axis',(0.,-1.,0.));
#27770=DIRECTION('ref_axis',(-0.154274306935522,0.,0.9880280553808));
#27771=DIRECTION('center_axis',(0.,1.,0.));
#27772=DIRECTION('ref_axis',(-0.154274306968473,0.,0.988028055375654));
#27773=DIRECTION('',(0.,-1.,0.));
#27774=DIRECTION('center_axis',(0.,-1.,0.));
#27775=DIRECTION('ref_axis',(-0.154274306968473,0.,0.988028055375654));
#27776=DIRECTION('',(0.,1.,0.));
#27777=DIRECTION('center_axis',(0.,-1.,0.));
#27778=DIRECTION('ref_axis',(0.581877193327017,0.,0.813276663802591));
#27779=DIRECTION('center_axis',(0.,-1.,0.));
#27780=DIRECTION('ref_axis',(0.581877193327157,0.,0.813276663802491));
#27781=DIRECTION('',(0.,1.,0.));
#27782=DIRECTION('center_axis',(0.,1.,0.));
#27783=DIRECTION('ref_axis',(0.581877193327157,0.,0.813276663802491));
#27784=DIRECTION('center_axis',(0.,-1.,0.));
#27785=DIRECTION('ref_axis',(0.994290944595386,0.,0.106702940426287));
#27786=DIRECTION('center_axis',(0.,1.,0.));
#27787=DIRECTION('ref_axis',(0.994290944591597,0.,0.106702940461588));
#27788=DIRECTION('',(0.,-1.,0.));
#27789=DIRECTION('center_axis',(0.,-1.,0.));
#27790=DIRECTION('ref_axis',(0.994290944591597,0.,0.106702940461588));
#27791=DIRECTION('center_axis',(0.772541698292714,0.,-0.634964033941301));
#27792=DIRECTION('ref_axis',(0.,-1.,0.));
#27793=DIRECTION('',(0.634964033941407,0.,0.772541698292626));
#27794=DIRECTION('',(0.,1.,0.));
#27795=DIRECTION('',(-0.634964033941407,0.,-0.772541698292626));
#27796=DIRECTION('center_axis',(0.,-1.,0.));
#27797=DIRECTION('ref_axis',(-0.0239909289777986,0.,0.999712176242133));
#27798=DIRECTION('center_axis',(0.,1.,0.));
#27799=DIRECTION('ref_axis',(-0.0239909290168162,0.,0.999712176241197));
#27800=DIRECTION('',(0.,-1.,0.));
#27801=DIRECTION('center_axis',(0.,-1.,0.));
#27802=DIRECTION('ref_axis',(-0.0239909290168162,0.,0.999712176241197));
#27803=DIRECTION('',(0.,1.,0.));
#27804=DIRECTION('center_axis',(0.,-1.,0.));
#27805=DIRECTION('ref_axis',(0.683053059422266,0.,0.730368754817649));
#27806=DIRECTION('center_axis',(0.,-1.,0.));
#27807=DIRECTION('ref_axis',(0.683053059422291,0.,0.730368754817625));
#27808=DIRECTION('',(0.,1.,0.));
#27809=DIRECTION('center_axis',(0.,1.,0.));
#27810=DIRECTION('ref_axis',(0.683053059422291,0.,0.730368754817625));
#27811=DIRECTION('center_axis',(0.,-1.,0.));
#27812=DIRECTION('ref_axis',(0.999712176242133,0.,-0.0239909289777986));
#27813=DIRECTION('center_axis',(0.,1.,0.));
#27814=DIRECTION('ref_axis',(0.999712176241197,0.,-0.0239909290168162));
#27815=DIRECTION('',(0.,-1.,0.));
#27816=DIRECTION('center_axis',(0.,-1.,0.));
#27817=DIRECTION('ref_axis',(0.999712176241197,0.,-0.0239909290168162));
#27818=DIRECTION('center_axis',(0.683053059422266,0.,-0.730368754817649));
#27819=DIRECTION('ref_axis',(0.,-1.,0.));
#27820=DIRECTION('',(0.730368754817616,0.,0.683053059422301));
#27821=DIRECTION('',(0.,1.,0.));
#27822=DIRECTION('',(-0.730368754817616,0.,-0.683053059422301));
#27823=DIRECTION('center_axis',(0.,-1.,0.));
#27824=DIRECTION('ref_axis',(0.106702940426287,0.,0.994290944595386));
#27825=DIRECTION('center_axis',(0.,1.,0.));
#27826=DIRECTION('ref_axis',(0.106702940461588,0.,0.994290944591597));
#27827=DIRECTION('',(0.,-1.,0.));
#27828=DIRECTION('center_axis',(0.,-1.,0.));
#27829=DIRECTION('ref_axis',(0.106702940461588,0.,0.994290944591597));
#27830=DIRECTION('',(0.,1.,0.));
#27831=DIRECTION('center_axis',(0.,-1.,0.));
#27832=DIRECTION('ref_axis',(0.772541698292714,0.,0.634964033941301));
#27833=DIRECTION('center_axis',(0.,-1.,0.));
#27834=DIRECTION('ref_axis',(0.772541698292649,0.,0.63496403394138));
#27835=DIRECTION('',(0.,1.,0.));
#27836=DIRECTION('center_axis',(0.,1.,0.));
#27837=DIRECTION('ref_axis',(0.772541698292649,0.,0.63496403394138));
#27838=DIRECTION('center_axis',(0.,-1.,0.));
#27839=DIRECTION('ref_axis',(0.988028055380798,0.,-0.15427430693553));
#27840=DIRECTION('center_axis',(0.,1.,0.));
#27841=DIRECTION('ref_axis',(0.988028055375653,0.,-0.154274306968481));
#27842=DIRECTION('',(0.,-1.,0.));
#27843=DIRECTION('center_axis',(0.,-1.,0.));
#27844=DIRECTION('ref_axis',(0.988028055375653,0.,-0.154274306968481));
#27845=DIRECTION('center_axis',(0.581877193327018,0.,-0.813276663802591));
#27846=DIRECTION('ref_axis',(0.,-1.,0.));
#27847=DIRECTION('',(0.813276663802457,0.,0.581877193327205));
#27848=DIRECTION('',(0.,1.,0.));
#27849=DIRECTION('',(-0.813276663802457,0.,-0.581877193327205));
#27850=DIRECTION('center_axis',(0.,-1.,0.));
#27851=DIRECTION('ref_axis',(0.235571092936033,0.,0.971857119217081));
#27852=DIRECTION('center_axis',(0.,1.,0.));
#27853=DIRECTION('ref_axis',(0.235571092964656,0.,0.971857119210143));
#27854=DIRECTION('',(0.,-1.,0.));
#27855=DIRECTION('center_axis',(0.,-1.,0.));
#27856=DIRECTION('ref_axis',(0.235571092964656,0.,0.971857119210143));
#27857=DIRECTION('',(0.,1.,0.));
#27858=DIRECTION('center_axis',(0.,-1.,0.));
#27859=DIRECTION('ref_axis',(0.848811934516349,0.,0.528694902398929));
#27860=DIRECTION('center_axis',(0.,-1.,0.));
#27861=DIRECTION('ref_axis',(0.848811934516223,0.,0.528694902399131));
#27862=DIRECTION('',(0.,1.,0.));
#27863=DIRECTION('center_axis',(0.,1.,0.));
#27864=DIRECTION('ref_axis',(0.848811934516223,0.,0.528694902399131));
#27865=DIRECTION('center_axis',(0.,-1.,0.));
#27866=DIRECTION('ref_axis',(0.959438500558773,0.,-0.28191800872866));
#27867=DIRECTION('center_axis',(0.,1.,0.));
#27868=DIRECTION('ref_axis',(0.959438500551133,0.,-0.281918008754661));
#27869=DIRECTION('',(0.,-1.,0.));
#27870=DIRECTION('center_axis',(0.,-1.,0.));
#27871=DIRECTION('ref_axis',(0.959438500551133,0.,-0.281918008754661));
#27872=DIRECTION('center_axis',(0.470745247127108,0.,-0.882269183586981));
#27873=DIRECTION('ref_axis',(0.,-1.,0.));
#27874=DIRECTION('',(0.882269183586787,0.,0.470745247127471));
#27875=DIRECTION('',(0.,1.,0.));
#27876=DIRECTION('',(-0.882269183586787,0.,-0.470745247127471));
#27877=DIRECTION('center_axis',(-0.528694902398929,0.,0.848811934516349));
#27878=DIRECTION('ref_axis',(0.,1.,0.));
#27879=DIRECTION('',(0.84881193451618,0.,0.528694902399201));
#27880=DIRECTION('',(0.,-1.,0.));
#27881=DIRECTION('',(-0.84881193451618,0.,-0.528694902399201));
#27882=DIRECTION('center_axis',(-0.634964033941301,0.,0.772541698292714));
#27883=DIRECTION('ref_axis',(0.,1.,0.));
#27884=DIRECTION('',(0.772541698292626,0.,0.634964033941407));
#27885=DIRECTION('',(0.,-1.,0.));
#27886=DIRECTION('',(-0.772541698292626,0.,-0.634964033941407));
#27887=DIRECTION('center_axis',(-0.813276663802591,0.,0.581877193327018));
#27888=DIRECTION('ref_axis',(0.,1.,0.));
#27889=DIRECTION('',(0.581877193327206,0.,0.813276663802456));
#27890=DIRECTION('',(0.,-1.,0.));
#27891=DIRECTION('',(-0.581877193327206,0.,-0.813276663802456));
#27892=DIRECTION('center_axis',(-0.882269183586981,0.,0.470745247127108));
#27893=DIRECTION('ref_axis',(0.,1.,0.));
#27894=DIRECTION('',(0.470745247127471,0.,0.882269183586787));
#27895=DIRECTION('',(0.,-1.,0.));
#27896=DIRECTION('',(-0.470745247127471,0.,-0.882269183586787));
#27897=DIRECTION('center_axis',(0.,1.,0.));
#27898=DIRECTION('ref_axis',(-0.430511096808295,0.,-0.902585284349861));
#27899=DIRECTION('center_axis',(0.,-1.,0.));
#27900=DIRECTION('ref_axis',(-0.430511096808622,0.,-0.902585284349705));
#27901=DIRECTION('',(0.,-1.,0.));
#27902=DIRECTION('center_axis',(0.,1.,0.));
#27903=DIRECTION('ref_axis',(-0.430511096808622,0.,-0.902585284349705));
#27904=DIRECTION('center_axis',(0.,1.,0.));
#27905=DIRECTION('ref_axis',(-0.430511096808295,0.,-0.902585284349861));
#27906=DIRECTION('center_axis',(0.,1.,0.));
#27907=DIRECTION('ref_axis',(-0.430511096808622,0.,-0.902585284349705));
#27908=DIRECTION('center_axis',(0.,-1.,0.));
#27909=DIRECTION('ref_axis',(-0.430511096808622,0.,-0.902585284349705));
#27910=DIRECTION('center_axis',(0.,1.,0.));
#27911=DIRECTION('ref_axis',(1.,0.,0.));
#27912=DIRECTION('',(0.902585284349658,0.,0.430511096808719));
#27913=DIRECTION('center_axis',(0.,-1.,0.));
#27914=DIRECTION('ref_axis',(0.430511096808602,0.,0.902585284349714));
#27915=DIRECTION('',(-0.430511096808721,0.,-0.902585284349657));
#27916=DIRECTION('center_axis',(0.,1.,0.));
#27917=DIRECTION('ref_axis',(-0.430511096808622,0.,-0.902585284349705));
#27918=DIRECTION('center_axis',(0.,1.,0.));
#27919=DIRECTION('ref_axis',(-0.430511096808622,0.,-0.902585284349705));
#27920=DIRECTION('center_axis',(0.,1.,0.));
#27921=DIRECTION('ref_axis',(-0.430511096808622,0.,-0.902585284349705));
#27922=DIRECTION('',(0.683053059422301,0.,0.730368754817616));
#27923=DIRECTION('center_axis',(0.,1.,0.));
#27924=DIRECTION('ref_axis',(-0.430511096808622,0.,-0.902585284349705));
#27925=DIRECTION('center_axis',(0.,1.,0.));
#27926=DIRECTION('ref_axis',(-0.430511096808295,0.,-0.902585284349861));
#27927=DIRECTION('center_axis',(0.,-1.,0.));
#27928=DIRECTION('ref_axis',(-0.430511096808622,0.,-0.902585284349705));
#27929=DIRECTION('',(0.,-1.,0.));
#27930=DIRECTION('center_axis',(0.,1.,0.));
#27931=DIRECTION('ref_axis',(-0.430511096808295,0.,-0.902585284349861));
#27932=DIRECTION('',(0.,1.,0.));
#27933=DIRECTION('center_axis',(0.,-1.,0.));
#27934=DIRECTION('ref_axis',(-0.430511096808622,0.,-0.902585284349705));
#27935=DIRECTION('center_axis',(-0.730368754817649,0.,0.683053059422266));
#27936=DIRECTION('ref_axis',(0.,1.,0.));
#27937=DIRECTION('',(-0.683053059422301,0.,-0.730368754817616));
#27938=DIRECTION('center_axis',(0.,1.,0.));
#27939=DIRECTION('ref_axis',(-0.430511096808295,0.,-0.902585284349861));
#27940=DIRECTION('center_axis',(0.,-1.,0.));
#27941=DIRECTION('ref_axis',(-0.430511096808622,0.,-0.902585284349705));
#27942=DIRECTION('center_axis',(0.430511096808293,0.,-0.902585284349862));
#27943=DIRECTION('ref_axis',(0.,-1.,0.));
#27944=DIRECTION('',(-0.902585284349658,0.,-0.430511096808719));
#27945=DIRECTION('',(0.,1.,0.));
#27946=DIRECTION('center_axis',(0.,1.,0.));
#27947=DIRECTION('ref_axis',(0.430511096808295,0.,0.902585284349861));
#27948=DIRECTION('center_axis',(0.,1.,0.));
#27949=DIRECTION('ref_axis',(0.430511096808602,0.,0.902585284349714));
#27950=DIRECTION('',(0.,1.,0.));
#27951=DIRECTION('center_axis',(-0.902585284349861,0.,0.430511096808295));
#27952=DIRECTION('ref_axis',(0.,1.,0.));
#27953=DIRECTION('',(0.430511096808721,0.,0.902585284349657));
#27954=DIRECTION('center_axis',(0.,1.,0.));
#27955=DIRECTION('ref_axis',(-0.430511096808295,0.,-0.902585284349861));
#27956=DIRECTION('center_axis',(0.,-1.,0.));
#27957=DIRECTION('ref_axis',(-0.430511096808622,0.,-0.902585284349705));
#27958=DIRECTION('center_axis',(0.,1.,0.));
#27959=DIRECTION('ref_axis',(1.,0.,0.));
#33932=CARTESIAN_POINT('',(0.,0.,0.));
#33933=CARTESIAN_POINT('Origin',(0.00643329000430773,-0.008,0.0115261780187742));
#33934=CARTESIAN_POINT('',(0.00621272270841098,-0.008,0.011643864330556));
#33935=CARTESIAN_POINT('',(0.00655513261802568,-0.008,0.0117444768448874));
#33936=CARTESIAN_POINT('Origin',(0.00643329000431773,-0.00799999999999,
0.0115261780187842));
#33937=CARTESIAN_POINT('',(0.00655513261802568,-0.024,0.0117444768448874));
#33938=CARTESIAN_POINT('',(0.00655513261803568,-0.00799999999999,0.0117444768448974));
#33939=CARTESIAN_POINT('',(0.00621272270841098,-0.024,0.011643864330556));
#33940=CARTESIAN_POINT('Origin',(0.00643329000431773,-0.02400000000001,
0.0115261780187842));
#33941=CARTESIAN_POINT('',(0.00621272270842098,-0.00799999999999,0.011643864330566));
#33942=CARTESIAN_POINT('Origin',(-4.44089209850063E-17,-0.008,6.72997231505748E-33));
#33943=CARTESIAN_POINT('',(0.00689344899281767,-0.008,0.0115491497948299));
#33944=CARTESIAN_POINT('Origin',(-4.44089209850063E-17,-0.00799999999999,
6.72997231505748E-33));
#33945=CARTESIAN_POINT('',(0.00689344899281767,-0.024,0.0115491497948299));
#33946=CARTESIAN_POINT('',(0.00689344899282767,-0.00799999999999,0.0115491497948399));
#33947=CARTESIAN_POINT('Origin',(-4.44089209850063E-17,-0.02400000000001,
6.72997231505748E-33));
#33948=CARTESIAN_POINT('Origin',(0.00676531797064634,-0.008,0.0113344815830301));
#33949=CARTESIAN_POINT('',(0.00697752095427542,-0.008,0.0112023078574304));
#33950=CARTESIAN_POINT('Origin',(0.00676531797065634,-0.00799999999999,
0.0113344815830401));
#33951=CARTESIAN_POINT('',(0.00697752095427542,-0.024,0.0112023078574304));
#33952=CARTESIAN_POINT('',(0.00697752095428542,-0.00799999999999,0.0112023078574404));
#33953=CARTESIAN_POINT('Origin',(0.00676531797065634,-0.02400000000001,
0.0113344815830401));
#33954=CARTESIAN_POINT('Origin',(0.00687303373118604,-0.008,0.0110345551487125));
#33955=CARTESIAN_POINT('',(0.00687303373118604,-0.008,0.0110345551487125));
#33956=CARTESIAN_POINT('',(0.00673974017575285,-0.00799999999999,0.0108205542946554));
#33957=CARTESIAN_POINT('',(0.00687303373118604,-0.024,0.0110345551487125));
#33958=CARTESIAN_POINT('',(0.00687303373119603,-0.016,0.0110345551487225));
#33959=CARTESIAN_POINT('',(0.00673974017575285,-0.02400000000001,0.0108205542946554));
#33960=CARTESIAN_POINT('Origin',(0.00788272044413945,-0.008,0.0105878571202838));
#33961=CARTESIAN_POINT('',(0.00767940127818881,-0.008,0.0107333264186156));
#33962=CARTESIAN_POINT('',(0.00803201439194512,-0.008,0.0107883847172589));
#33963=CARTESIAN_POINT('Origin',(0.00788272044414944,-0.00799999999999,
0.0105878571202938));
#33964=CARTESIAN_POINT('',(0.00803201439194512,-0.024,0.0107883847172589));
#33965=CARTESIAN_POINT('',(0.00803201439195513,-0.00799999999999,0.0107883847172689));
#33966=CARTESIAN_POINT('',(0.00767940127818881,-0.024,0.0107333264186156));
#33967=CARTESIAN_POINT('Origin',(0.00788272044414944,-0.02400000000001,
0.0105878571202938));
#33968=CARTESIAN_POINT('',(0.00767940127819881,-0.00799999999999,0.0107333264186256));
#33969=CARTESIAN_POINT('Origin',(-4.44089209850063E-17,-0.008,6.72997231505748E-33));
#33970=CARTESIAN_POINT('',(0.00834194112716969,-0.008,0.0105505695690249));
#33971=CARTESIAN_POINT('Origin',(-4.44089209850063E-17,-0.00799999999999,
6.72997231505748E-33));
#33972=CARTESIAN_POINT('',(0.00834194112716969,-0.024,0.0105505695690249));
#33973=CARTESIAN_POINT('',(0.00834194112717969,-0.00799999999999,0.0105505695690349));
#33974=CARTESIAN_POINT('Origin',(-4.44089209850063E-17,-0.02400000000001,
6.72997231505748E-33));
#33975=CARTESIAN_POINT('Origin',(0.00818688645937843,-0.008,0.010354462327965));
#33976=CARTESIAN_POINT('',(0.0083800218839516,-0.008,0.0101957213194796));
#33977=CARTESIAN_POINT('Origin',(0.00818688645938842,-0.00799999999999,
0.010354462327975));
#33978=CARTESIAN_POINT('',(0.0083800218839516,-0.024,0.0101957213194796));
#33979=CARTESIAN_POINT('',(0.00838002188396161,-0.00799999999999,0.0101957213194896));
#33980=CARTESIAN_POINT('Origin',(0.00818688645938842,-0.02400000000001,
0.010354462327975));
#33981=CARTESIAN_POINT('Origin',(0.00825453244123688,-0.008,0.0100430420778053));
#33982=CARTESIAN_POINT('',(0.00825453244123688,-0.008,0.0100430420778053));
#33983=CARTESIAN_POINT('',(0.00818084247458016,-0.00799999999999,0.0099533857052449));
#33984=CARTESIAN_POINT('',(0.00825453244123688,-0.024,0.0100430420778053));
#33985=CARTESIAN_POINT('',(0.00825453244124687,-0.016,0.0100430420778153));
#33986=CARTESIAN_POINT('',(0.00818084247458016,-0.02400000000001,0.0099533857052449));
#33987=CARTESIAN_POINT('Origin',(0.00919727535166895,-0.008,0.00946837505095685));
#33988=CARTESIAN_POINT('',(0.00901468316296453,-0.008,0.00963913831581242));
#33989=CARTESIAN_POINT('',(0.00937146617272329,-0.008,0.00964770033601285));
#33990=CARTESIAN_POINT('Origin',(0.00919727535167895,-0.00799999999999,
0.00946837505096685));
#33991=CARTESIAN_POINT('',(0.00937146617272329,-0.024,0.00964770033601285));
#33992=CARTESIAN_POINT('',(0.00937146617273328,-0.00799999999999,0.00964770033602285));
#33993=CARTESIAN_POINT('',(0.00901468316296453,-0.024,0.00963913831581242));
#33994=CARTESIAN_POINT('Origin',(0.00919727535167895,-0.02400000000001,
0.00946837505096685));
#33995=CARTESIAN_POINT('',(0.00901468316297454,-0.00799999999999,0.00963913831582242));
#33996=CARTESIAN_POINT('Origin',(-4.44089209850063E-17,-0.008,6.72997231505748E-33));
#33997=CARTESIAN_POINT('',(0.0096477003360128,-0.008,0.00937146617272333));
#33998=CARTESIAN_POINT('Origin',(-4.44089209850063E-17,-0.00799999999999,
6.72997231505748E-33));
#33999=CARTESIAN_POINT('',(0.0096477003360128,-0.024,0.00937146617272333));
#34000=CARTESIAN_POINT('',(0.00964770033602281,-0.00799999999999,0.00937146617273333));
#34001=CARTESIAN_POINT('Origin',(-4.44089209850063E-17,-0.02400000000001,
6.72997231505748E-33));
#34002=CARTESIAN_POINT('Origin',(0.0094683750509568,-0.008,0.00919727535166899));
#34003=CARTESIAN_POINT('',(0.00963913831581237,-0.008,0.00901468316296458));
#34004=CARTESIAN_POINT('Origin',(0.0094683750509668,-0.00799999999999,0.00919727535167899));
#34005=CARTESIAN_POINT('',(0.00963913831581237,-0.024,0.00901468316296458));
#34006=CARTESIAN_POINT('',(0.00963913831582238,-0.00799999999999,0.00901468316297458));
#34007=CARTESIAN_POINT('Origin',(0.0094683750509668,-0.02400000000001,0.00919727535167899));
#34008=CARTESIAN_POINT('Origin',(0.00949479381262939,-0.008,0.00887968977248946));
#34009=CARTESIAN_POINT('',(0.00949479381262939,-0.008,0.00887968977248946));
#34010=CARTESIAN_POINT('',(0.00942962993438202,-0.00799999999999,0.00881874742507027));
#34011=CARTESIAN_POINT('',(0.00949479381262939,-0.024,0.00887968977248946));
#34012=CARTESIAN_POINT('',(0.00949479381263939,-0.016,0.00887968977249946));
#34013=CARTESIAN_POINT('',(0.00942962993438202,-0.02400000000001,0.00881874742507027));
#34014=CARTESIAN_POINT('Origin',(0.010354462327965,-0.008,0.00818688645937847));
#34015=CARTESIAN_POINT('',(0.0101957213194795,-0.008,0.00838002188395165));
#34016=CARTESIAN_POINT('',(0.0105505695690249,-0.008,0.00834194112716973));
#34017=CARTESIAN_POINT('Origin',(0.010354462327975,-0.00799999999999,0.00818688645938847));
#34018=CARTESIAN_POINT('',(0.0105505695690249,-0.024,0.00834194112716973));
#34019=CARTESIAN_POINT('',(0.0105505695690349,-0.00799999999999,0.00834194112717973));
#34020=CARTESIAN_POINT('',(0.0101957213194795,-0.024,0.00838002188395165));
#34021=CARTESIAN_POINT('Origin',(0.010354462327975,-0.02400000000001,0.00818688645938847));
#34022=CARTESIAN_POINT('',(0.0101957213194895,-0.00799999999999,0.00838002188396165));
#34023=CARTESIAN_POINT('Origin',(-4.44089209850063E-17,-0.008,6.72997231505748E-33));
#34024=CARTESIAN_POINT('',(0.0107883847172589,-0.008,0.00803201439194517));
#34025=CARTESIAN_POINT('Origin',(-4.44089209850063E-17,-0.00799999999999,
6.72997231505748E-33));
#34026=CARTESIAN_POINT('',(0.0107883847172589,-0.024,0.00803201439194517));
#34027=CARTESIAN_POINT('',(0.0107883847172689,-0.00799999999999,0.00803201439195516));
#34028=CARTESIAN_POINT('Origin',(-4.44089209850063E-17,-0.02400000000001,
6.72997231505748E-33));
#34029=CARTESIAN_POINT('Origin',(0.0105878571202839,-0.008,0.00788272044413949));
#34030=CARTESIAN_POINT('',(0.0107333264186156,-0.008,0.00767940127818885));
#34031=CARTESIAN_POINT('Origin',(0.0105878571202939,-0.00799999999999,0.00788272044414949));
#34032=CARTESIAN_POINT('',(0.0107333264186156,-0.024,0.00767940127818885));
#34033=CARTESIAN_POINT('',(0.0107333264186256,-0.00799999999999,0.00767940127819885));
#34034=CARTESIAN_POINT('Origin',(0.0105878571202939,-0.02400000000001,0.00788272044414949));
#34035=CARTESIAN_POINT('Origin',(0.0105725966294337,-0.008,0.00756440351325123));
#34036=CARTESIAN_POINT('',(0.0105725966294337,-0.008,0.00756440351325123));
#34037=CARTESIAN_POINT('',(0.0104326500269425,-0.00799999999999,0.00746427554955177));
#34038=CARTESIAN_POINT('',(0.0105725966294337,-0.024,0.00756440351325123));
#34039=CARTESIAN_POINT('',(0.0105725966294436,-0.016,0.00756440351326123));
#34040=CARTESIAN_POINT('',(0.0104326500269425,-0.02400000000001,0.00746427554955177));
#34041=CARTESIAN_POINT('Origin',(0.0113344815830301,-0.008,0.00676531797064638));
#34042=CARTESIAN_POINT('',(0.0112023078574304,-0.008,0.00697752095427547));
#34043=CARTESIAN_POINT('',(0.0115491497948299,-0.008,0.00689344899281771));
#34044=CARTESIAN_POINT('Origin',(0.0113344815830401,-0.00799999999999,0.00676531797065638));
#34045=CARTESIAN_POINT('',(0.0115491497948299,-0.024,0.00689344899281771));
#34046=CARTESIAN_POINT('',(0.0115491497948398,-0.00799999999999,0.00689344899282771));
#34047=CARTESIAN_POINT('',(0.0112023078574304,-0.024,0.00697752095427547));
#34048=CARTESIAN_POINT('Origin',(0.0113344815830401,-0.02400000000001,0.00676531797065638));
#34049=CARTESIAN_POINT('',(0.0112023078574404,-0.00799999999999,0.00697752095428547));
#34050=CARTESIAN_POINT('Origin',(-4.44089209850063E-17,-0.008,6.72997231505748E-33));
#34051=CARTESIAN_POINT('',(0.0117444768448874,-0.008,0.00655513261802572));
#34052=CARTESIAN_POINT('Origin',(-4.44089209850063E-17,-0.00799999999999,
6.72997231505748E-33));
#34053=CARTESIAN_POINT('',(0.0117444768448874,-0.024,0.00655513261802572));
#34054=CARTESIAN_POINT('',(0.0117444768448974,-0.00799999999999,0.00655513261803572));
#34055=CARTESIAN_POINT('Origin',(-4.44089209850063E-17,-0.02400000000001,
6.72997231505748E-33));
#34056=CARTESIAN_POINT('Origin',(0.0115261780187742,-0.008,0.00643329000430777));
#34057=CARTESIAN_POINT('',(0.011643864330556,-0.008,0.00621272270841103));
#34058=CARTESIAN_POINT('Origin',(0.0115261780187842,-0.00799999999999,0.00643329000431777));
#34059=CARTESIAN_POINT('',(0.011643864330556,-0.024,0.00621272270841103));
#34060=CARTESIAN_POINT('',(0.011643864330566,-0.00799999999999,0.00621272270842103));
#34061=CARTESIAN_POINT('Origin',(0.0115261780187842,-0.02400000000001,0.00643329000431777));
#34062=CARTESIAN_POINT('Origin',(0.0114694993866308,-0.008,0.0061196882126524));
#34063=CARTESIAN_POINT('',(0.0114694993866308,-0.008,0.0061196882126524));
#34064=CARTESIAN_POINT('',(0.0111490530784194,-0.00799999999999,0.00594871026243939));
#34065=CARTESIAN_POINT('',(0.0114694993866308,-0.024,0.0061196882126524));
#34066=CARTESIAN_POINT('',(0.0114694993866408,-0.016,0.0061196882126624));
#34067=CARTESIAN_POINT('',(0.0111490530784194,-0.02400000000001,0.00594871026243939));
#34068=CARTESIAN_POINT('Origin',(0.0114165205192449,-0.008,0.00711094643726559));
#34069=CARTESIAN_POINT('',(0.0110345551487124,-0.024,0.00687303373118608));
#34070=CARTESIAN_POINT('',(0.0110115369799215,-0.02400000000001,0.00685869652879265));
#34071=CARTESIAN_POINT('',(0.0110345551487124,-0.008,0.00687303373118608));
#34072=CARTESIAN_POINT('',(0.0110345551487224,-0.016,0.00687303373119607));
#34073=CARTESIAN_POINT('',(0.0110115369799215,-0.00799999999999,0.00685869652879265));
#34074=CARTESIAN_POINT('Origin',(0.010390685842037,-0.008,0.0085402662565105));
#34075=CARTESIAN_POINT('',(0.0100430420778052,-0.024,0.00825453244123691));
#34076=CARTESIAN_POINT('',(0.0101272075873608,-0.02400000000001,0.008323709382217));
#34077=CARTESIAN_POINT('',(0.0100430420778052,-0.008,0.00825453244123691));
#34078=CARTESIAN_POINT('',(0.0100430420778153,-0.016,0.00825453244124691));
#34079=CARTESIAN_POINT('',(0.0101272075873608,-0.00799999999999,0.008323709382217));
#34080=CARTESIAN_POINT('Origin',(0.00782624825024835,-0.008,0.0109385711281449));
#34081=CARTESIAN_POINT('',(0.00756440351325119,-0.024,0.0105725966294337));
#34082=CARTESIAN_POINT('',(0.00759519791805031,-0.02400000000001,0.0106156372762982));
#34083=CARTESIAN_POINT('',(0.00756440351325119,-0.008,0.0105725966294337));
#34084=CARTESIAN_POINT('',(0.00756440351326119,-0.016,0.0105725966294437));
#34085=CARTESIAN_POINT('',(0.00759519791805031,-0.00799999999999,0.0106156372762982));
#34086=CARTESIAN_POINT('Origin',(0.00633152357385956,-0.008,0.0118665205192449));
#34087=CARTESIAN_POINT('',(0.00611968821265236,-0.024,0.0114694993866308));
#34088=CARTESIAN_POINT('',(0.00605462794304295,-0.02400000000001,0.0113475636447265));
#34089=CARTESIAN_POINT('',(0.00611968821265236,-0.008,0.0114694993866308));
#34090=CARTESIAN_POINT('',(0.00611968821266236,-0.016,0.0114694993866408));
#34091=CARTESIAN_POINT('',(0.00605462794304295,-0.00799999999999,0.0113475636447265));
#34092=CARTESIAN_POINT('Origin',(-4.44089209850063E-17,-0.016,6.72997231505748E-33));
#34093=CARTESIAN_POINT('',(0.0117336086965482,-0.008,0.00559664425850784));
#34094=CARTESIAN_POINT('Origin',(-4.44089209850063E-17,-0.00799999999999,
6.72997231505748E-33));
#34095=CARTESIAN_POINT('',(0.0117336086965482,-0.024,0.00559664425850784));
#34096=CARTESIAN_POINT('',(0.0117336086965582,-0.016,0.00559664425851784));
#34097=CARTESIAN_POINT('Origin',(-4.44089209850063E-17,-0.02400000000001,
6.72997231505748E-33));
#34098=CARTESIAN_POINT('Origin',(-4.44089209850063E-17,-0.016,6.72997231505748E-33));
#34099=CARTESIAN_POINT('Origin',(-4.44089209850063E-17,-0.02400000000001,
6.72997231505748E-33));
#34100=CARTESIAN_POINT('Origin',(-4.44089209850063E-17,-0.00799999999999,
6.72997231505748E-33));
#34101=CARTESIAN_POINT('Origin',(0.00907128985548541,-0.024,0.00907128985548545));
#34102=CARTESIAN_POINT('',(0.0125459354524631,-0.024,0.0059841042456353));
#34103=CARTESIAN_POINT('',(0.0125459354524731,-0.02400000000001,0.0059841042456453));
#34104=CARTESIAN_POINT('',(0.00598410424563526,-0.024,0.0125459354524631));
#34105=CARTESIAN_POINT('Origin',(-4.44089209850063E-17,-0.02400000000001,
6.72997231505748E-33));
#34106=CARTESIAN_POINT('',(0.0055966442585078,-0.024,0.0117336086965482));
#34107=CARTESIAN_POINT('',(0.0055966442585178,-0.02400000000001,0.0117336086965582));
#34108=CARTESIAN_POINT('Origin',(-4.44089209850063E-17,-0.02400000000001,
6.72997231505748E-33));
#34109=CARTESIAN_POINT('Origin',(-4.44089209850063E-17,-0.02400000000001,
6.72997231505748E-33));
#34110=CARTESIAN_POINT('',(0.00887968977248941,-0.024,0.00949479381262943));
#34111=CARTESIAN_POINT('Origin',(-4.44089209850063E-17,-0.02400000000001,
6.72997231505748E-33));
#34112=CARTESIAN_POINT('',(0.00897243436344023,-0.02400000000001,0.00959396290421603));
#34113=CARTESIAN_POINT('Origin',(-4.44089209850063E-17,-0.02400000000001,
6.72997231505748E-33));
#34114=CARTESIAN_POINT('Origin',(-4.44089209850063E-17,-0.016,6.72997231505748E-33));
#34115=CARTESIAN_POINT('',(0.00887968977248941,-0.008,0.00949479381262943));
#34116=CARTESIAN_POINT('Origin',(-4.44089209850063E-17,-0.00799999999999,
6.72997231505748E-33));
#34117=CARTESIAN_POINT('',(0.00887968977249942,-0.016,0.00949479381263943));
#34118=CARTESIAN_POINT('Origin',(-4.44089209850063E-17,-0.016,6.72997231505748E-33));
#34119=CARTESIAN_POINT('',(0.0055966442585078,-0.008,0.0117336086965482));
#34120=CARTESIAN_POINT('',(0.0055966442585178,-0.016,0.0117336086965582));
#34121=CARTESIAN_POINT('Origin',(-4.44089209850063E-17,-0.00799999999999,
6.72997231505748E-33));
#34122=CARTESIAN_POINT('Origin',(0.00918706364922943,-0.008,0.00982345975229737));
#34123=CARTESIAN_POINT('',(0.00897243436344023,-0.00799999999999,0.00959396290421603));
#34124=CARTESIAN_POINT('Origin',(-4.44089209850063E-17,-0.016,6.72997231505748E-33));
#34125=CARTESIAN_POINT('Origin',(-4.44089209850063E-17,-0.00799999999999,
6.72997231505748E-33));
#34126=CARTESIAN_POINT('Origin',(0.0125459354524631,-0.016,0.0059841042456353));
#34127=CARTESIAN_POINT('',(0.0125459354524631,-0.008,0.0059841042456353));
#34128=CARTESIAN_POINT('',(0.0125459354524731,-0.00799999999999,0.0059841042456453));
#34129=CARTESIAN_POINT('',(0.0125459354524731,-0.016,0.0059841042456453));
#34130=CARTESIAN_POINT('Origin',(-4.44089209850063E-17,-0.016,6.72997231505748E-33));
#34131=CARTESIAN_POINT('',(0.00598410424563526,-0.008,0.0125459354524631));
#34132=CARTESIAN_POINT('Origin',(-4.44089209850063E-17,-0.00799999999999,
6.72997231505748E-33));
#34133=CARTESIAN_POINT('',(0.00598410424564526,-0.016,0.0125459354524731));
#34134=CARTESIAN_POINT('Origin',(0.0055966442585078,-0.016,0.0117336086965482));
#34135=CARTESIAN_POINT('',(0.0055966442585178,-0.00799999999999,0.0117336086965582));
#34136=CARTESIAN_POINT('Origin',(-4.44089209850063E-17,-0.016,6.72997231505748E-33));
#34137=CARTESIAN_POINT('Origin',(-4.44089209850063E-17,-0.00799999999999,
6.72997231505748E-33));
#34138=CARTESIAN_POINT('Origin',(0.00907128985548541,-0.008,0.00907128985548545));
#34836=UNCERTAINTY_MEASURE_WITH_UNIT(LENGTH_MEASURE(1.E-5),#34877,
'DISTANCE_ACCURACY_VALUE',
'Maximum model space distance between geometric entities at asserted c
onnectivities');
#34841=UNCERTAINTY_MEASURE_WITH_UNIT(LENGTH_MEASURE(1.E-5),#34877,
'DISTANCE_ACCURACY_VALUE',
'Maximum model space distance between geometric entities at asserted c
onnectivities');
#34871=(
GEOMETRIC_REPRESENTATION_CONTEXT(3)
GLOBAL_UNCERTAINTY_ASSIGNED_CONTEXT((#34836))
GLOBAL_UNIT_ASSIGNED_CONTEXT((#34877,#34878,#34879))
REPRESENTATION_CONTEXT('','3D')
);
#34876=(
GEOMETRIC_REPRESENTATION_CONTEXT(3)
GLOBAL_UNCERTAINTY_ASSIGNED_CONTEXT((#34841))
GLOBAL_UNIT_ASSIGNED_CONTEXT((#34877,#34878,#34879))
REPRESENTATION_CONTEXT('','3D')
);
#34877=(
LENGTH_UNIT()
NAMED_UNIT(*)
SI_UNIT($,.METRE.)
);
#34878=(
NAMED_UNIT(*)
PLANE_ANGLE_UNIT()
SI_UNIT($,.RADIAN.)
);
#34879=(
NAMED_UNIT(*)
SI_UNIT($,.STERADIAN.)
SOLID_ANGLE_UNIT()
);
#34909=SHAPE_DEFINITION_REPRESENTATION(#34943,#35013);
#34943=PRODUCT_DEFINITION_SHAPE('',$,#35048);
#35013=SHAPE_REPRESENTATION('',(#21968),#34871);
#35018=PRODUCT_DEFINITION_CONTEXT('part definition',#35122,'design');
#35048=PRODUCT_DEFINITION('Motor Stator Face 7','Motor Stator Face 7',#35082,
#35018);
#35082=PRODUCT_DEFINITION_FORMATION('',$,#35153);
#35122=APPLICATION_CONTEXT('Managed model based 3d engineering');
#35123=PRODUCT_CONTEXT('part definition',#35122,'mechanical');
#35153=PRODUCT('Motor Stator Face 7','Motor Stator Face 7',
'LEGAL AND USAGE DISCLAIMER: this Data/Model is provided \X2\201C\X0\A
S IS\X2\201D\X0\ for informational and representational only. It is a 
geometric approximation and is NOT engineered, certified, or guarantee
d for dimensional accuracy, exact tolerances, or production-level prec
ision. Vendor disclaims all implied warranties including fitness for a
 particular purpose. DO NOT USE FOR DIRECT PHYSICAL MANUFACTURING, AUT
OMATED PRODUCTION, OR SAFETY-CRITICAL SYSTEMS without independent engi
neering verification and resolution of any design discrepancies.',(#35123));
#35162=PRESENTATION_STYLE_ASSIGNMENT((#35171));
#35171=SURFACE_STYLE_USAGE(.BOTH.,#35180);
#35180=SURFACE_SIDE_STYLE('',(#35189));
#35189=SURFACE_STYLE_FILL_AREA(#35198);
#35198=FILL_AREA_STYLE('Aluminum - Anodized Glossy (Grey)',(#35207));
#35207=FILL_AREA_STYLE_COLOUR('Aluminum - Anodized Glossy (Grey)',#35216);
#35216=COLOUR_RGB('Aluminum - Anodized Glossy (Grey)',0.537254901960784,
0.537254901960784,0.537254901960784);
ENDSEC;
END-ISO-10303-21;
